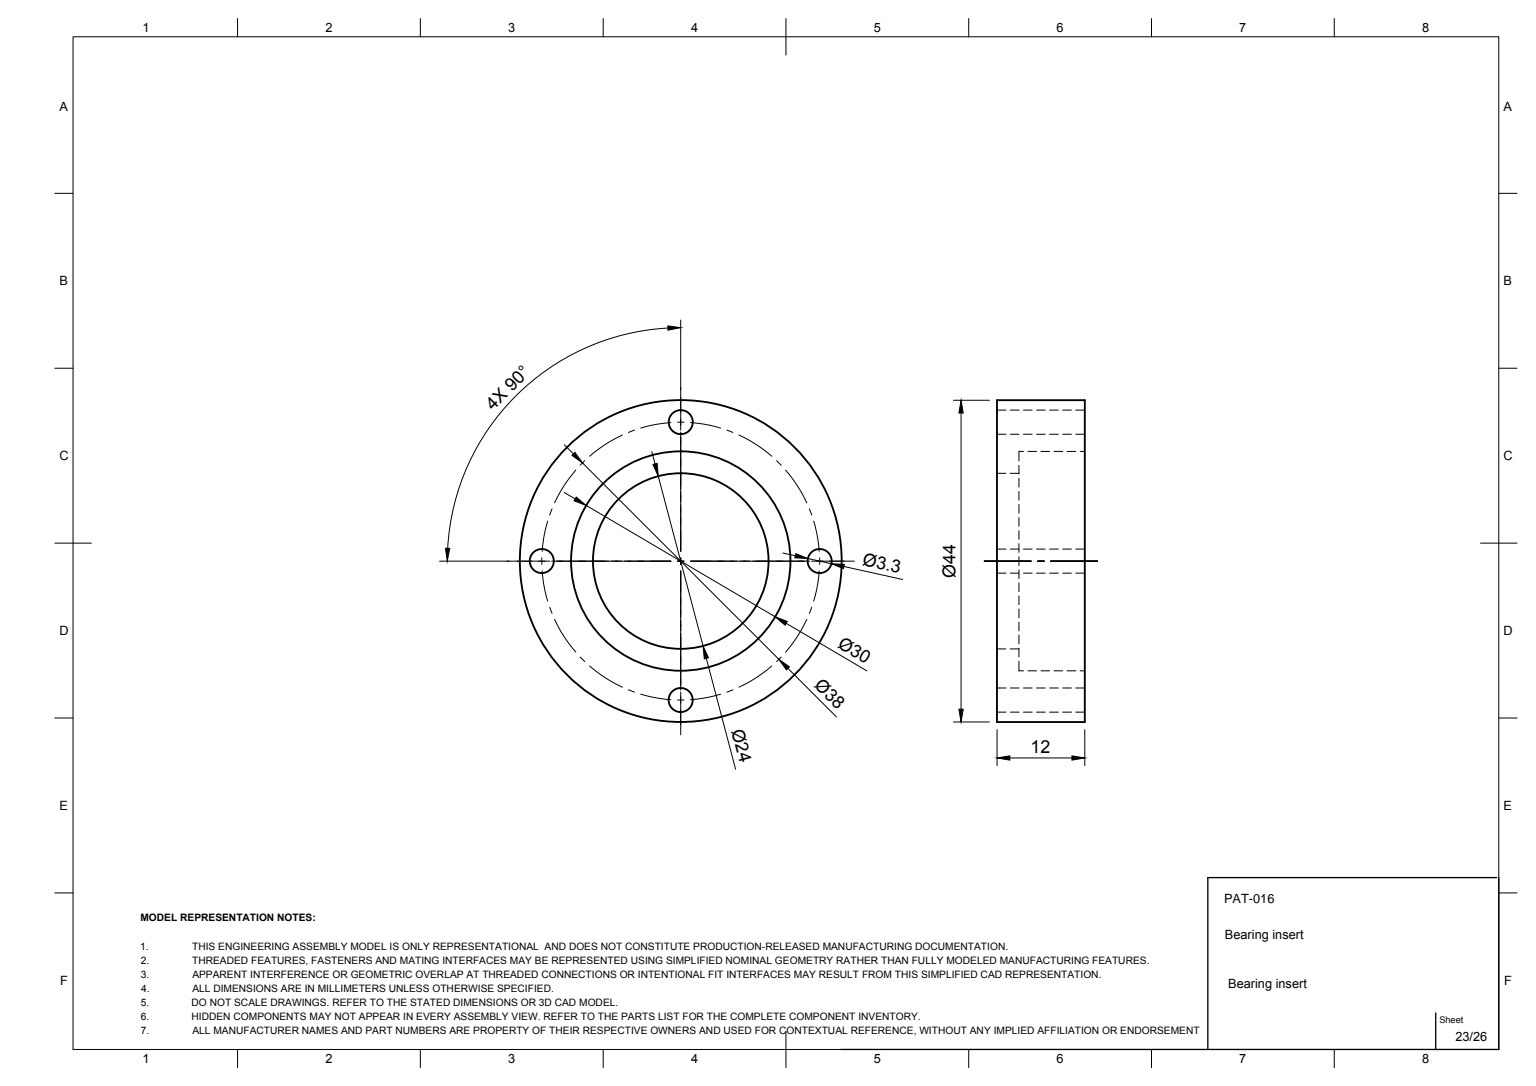
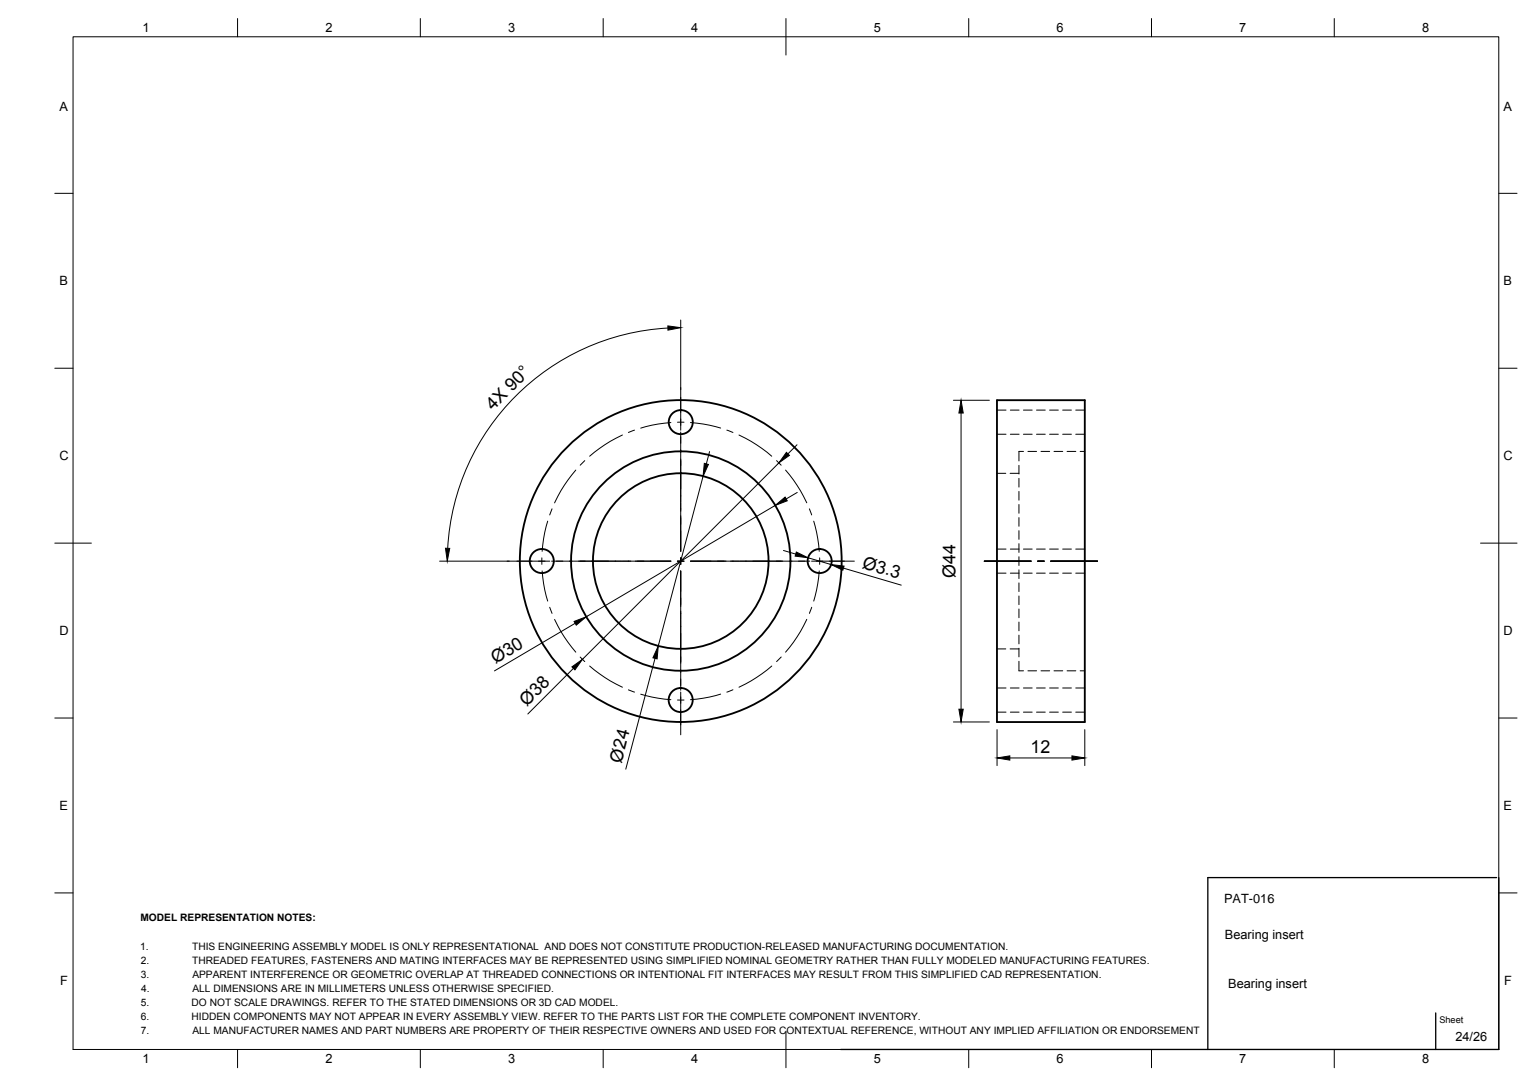
ISO-10303-21;
HEADER;
/* Generated by software containing ST-Developer
 * from STEP Tools, Inc. (www.steptools.com) 
 */

FILE_DESCRIPTION(
/* description */ ('Bracket-mounted idler roller'),
/* implementation_level */ '2;1');

FILE_NAME(
/* name */ 'Bearing insert.step',
/* time_stamp */ '2026-10-28T03:26:42-07:00',
/* author */ (''),
/* organization */ (''),
/* preprocessor_version */ 'ST-DEVELOPER v20.2',
/* originating_system */ 'Autodesk Translation Framework v15.17.0.0',
/* authorisation */ '');

FILE_SCHEMA (('AUTOMOTIVE_DESIGN { 1 0 10303 214 3 1 1 }'));
ENDSEC;

DATA;
#10=MECHANICAL_DESIGN_GEOMETRIC_PRESENTATION_REPRESENTATION('',(#304),#6241);
#254=SHAPE_REPRESENTATION_RELATIONSHIP('SRR','None',#6360,#275);
#275=ADVANCED_BREP_SHAPE_REPRESENTATION('',(#332),#6236);
#304=STYLED_ITEM('',(#6538),#332);
#332=MANIFOLD_SOLID_BREP('Body1',#3207);
#382=FACE_BOUND('',#901,.T.);
#383=FACE_BOUND('',#905,.T.);
#384=FACE_BOUND('',#906,.T.);
#385=FACE_BOUND('',#907,.T.);
#386=FACE_BOUND('',#908,.T.);
#387=FACE_BOUND('',#909,.T.);
#388=FACE_BOUND('',#911,.T.);
#389=FACE_BOUND('',#912,.T.);
#390=FACE_BOUND('',#913,.T.);
#391=FACE_BOUND('',#914,.T.);
#392=FACE_BOUND('',#915,.T.);
#495=PLANE('',#3757);
#496=PLANE('',#3764);
#497=PLANE('',#3765);
#658=FACE_OUTER_BOUND('',#895,.T.);
#659=FACE_OUTER_BOUND('',#896,.T.);
#660=FACE_OUTER_BOUND('',#897,.T.);
#661=FACE_OUTER_BOUND('',#898,.T.);
#662=FACE_OUTER_BOUND('',#899,.T.);
#663=FACE_OUTER_BOUND('',#900,.T.);
#664=FACE_OUTER_BOUND('',#902,.T.);
#665=FACE_OUTER_BOUND('',#903,.T.);
#666=FACE_OUTER_BOUND('',#904,.T.);
#667=FACE_OUTER_BOUND('',#910,.T.);
#895=EDGE_LOOP('',(#2732,#2733,#2734,#2735));
#896=EDGE_LOOP('',(#2736,#2737,#2738,#2739));
#897=EDGE_LOOP('',(#2740,#2741,#2742,#2743));
#898=EDGE_LOOP('',(#2744,#2745,#2746,#2747));
#899=EDGE_LOOP('',(#2748,#2749,#2750,#2751));
#900=EDGE_LOOP('',(#2752));
#901=EDGE_LOOP('',(#2753));
#902=EDGE_LOOP('',(#2754,#2755,#2756,#2757));
#903=EDGE_LOOP('',(#2758,#2759,#2760,#2761));
#904=EDGE_LOOP('',(#2762));
#905=EDGE_LOOP('',(#2763));
#906=EDGE_LOOP('',(#2764));
#907=EDGE_LOOP('',(#2765));
#908=EDGE_LOOP('',(#2766));
#909=EDGE_LOOP('',(#2767));
#910=EDGE_LOOP('',(#2768));
#911=EDGE_LOOP('',(#2769));
#912=EDGE_LOOP('',(#2770));
#913=EDGE_LOOP('',(#2771));
#914=EDGE_LOOP('',(#2772));
#915=EDGE_LOOP('',(#2773));
#1115=LINE('',#5940,#1297);
#1116=LINE('',#5946,#1298);
#1117=LINE('',#5952,#1299);
#1118=LINE('',#5958,#1300);
#1119=LINE('',#5964,#1301);
#1120=LINE('',#5971,#1302);
#1121=LINE('',#5977,#1303);
#1297=VECTOR('',#4620,0.165);
#1298=VECTOR('',#4627,0.165);
#1299=VECTOR('',#4634,0.165);
#1300=VECTOR('',#4641,0.165);
#1301=VECTOR('',#4648,1.2);
#1302=VECTOR('',#4657,1.5);
#1303=VECTOR('',#4664,2.2);
#1472=CIRCLE('',#3743,0.165);
#1473=CIRCLE('',#3744,0.165);
#1474=CIRCLE('',#3746,0.165);
#1475=CIRCLE('',#3747,0.165);
#1476=CIRCLE('',#3749,0.165);
#1477=CIRCLE('',#3750,0.165);
#1478=CIRCLE('',#3752,0.165);
#1479=CIRCLE('',#3753,0.165);
#1480=CIRCLE('',#3755,1.2);
#1481=CIRCLE('',#3756,1.2);
#1482=CIRCLE('',#3758,1.5);
#1483=CIRCLE('',#3760,1.5);
#1484=CIRCLE('',#3762,2.2);
#1485=CIRCLE('',#3763,2.2);
#1721=VERTEX_POINT('',#5937);
#1722=VERTEX_POINT('',#5939);
#1723=VERTEX_POINT('',#5943);
#1724=VERTEX_POINT('',#5945);
#1725=VERTEX_POINT('',#5949);
#1726=VERTEX_POINT('',#5951);
#1727=VERTEX_POINT('',#5955);
#1728=VERTEX_POINT('',#5957);
#1729=VERTEX_POINT('',#5961);
#1730=VERTEX_POINT('',#5963);
#1731=VERTEX_POINT('',#5967);
#1732=VERTEX_POINT('',#5970);
#1733=VERTEX_POINT('',#5974);
#1734=VERTEX_POINT('',#5976);
#2068=EDGE_CURVE('',#1721,#1721,#1472,.T.);
#2069=EDGE_CURVE('',#1721,#1722,#1115,.T.);
#2070=EDGE_CURVE('',#1722,#1722,#1473,.T.);
#2071=EDGE_CURVE('',#1723,#1723,#1474,.T.);
#2072=EDGE_CURVE('',#1723,#1724,#1116,.T.);
#2073=EDGE_CURVE('',#1724,#1724,#1475,.T.);
#2074=EDGE_CURVE('',#1725,#1725,#1476,.T.);
#2075=EDGE_CURVE('',#1725,#1726,#1117,.T.);
#2076=EDGE_CURVE('',#1726,#1726,#1477,.T.);
#2077=EDGE_CURVE('',#1727,#1727,#1478,.T.);
#2078=EDGE_CURVE('',#1727,#1728,#1118,.T.);
#2079=EDGE_CURVE('',#1728,#1728,#1479,.T.);
#2080=EDGE_CURVE('',#1729,#1729,#1480,.T.);
#2081=EDGE_CURVE('',#1729,#1730,#1119,.T.);
#2082=EDGE_CURVE('',#1730,#1730,#1481,.T.);
#2083=EDGE_CURVE('',#1731,#1731,#1482,.T.);
#2084=EDGE_CURVE('',#1731,#1732,#1120,.T.);
#2085=EDGE_CURVE('',#1732,#1732,#1483,.T.);
#2086=EDGE_CURVE('',#1733,#1733,#1484,.T.);
#2087=EDGE_CURVE('',#1733,#1734,#1121,.T.);
#2088=EDGE_CURVE('',#1734,#1734,#1485,.T.);
#2732=ORIENTED_EDGE('',*,*,#2068,.F.);
#2733=ORIENTED_EDGE('',*,*,#2069,.T.);
#2734=ORIENTED_EDGE('',*,*,#2070,.F.);
#2735=ORIENTED_EDGE('',*,*,#2069,.F.);
#2736=ORIENTED_EDGE('',*,*,#2071,.F.);
#2737=ORIENTED_EDGE('',*,*,#2072,.T.);
#2738=ORIENTED_EDGE('',*,*,#2073,.F.);
#2739=ORIENTED_EDGE('',*,*,#2072,.F.);
#2740=ORIENTED_EDGE('',*,*,#2074,.F.);
#2741=ORIENTED_EDGE('',*,*,#2075,.T.);
#2742=ORIENTED_EDGE('',*,*,#2076,.F.);
#2743=ORIENTED_EDGE('',*,*,#2075,.F.);
#2744=ORIENTED_EDGE('',*,*,#2077,.F.);
#2745=ORIENTED_EDGE('',*,*,#2078,.T.);
#2746=ORIENTED_EDGE('',*,*,#2079,.F.);
#2747=ORIENTED_EDGE('',*,*,#2078,.F.);
#2748=ORIENTED_EDGE('',*,*,#2080,.F.);
#2749=ORIENTED_EDGE('',*,*,#2081,.T.);
#2750=ORIENTED_EDGE('',*,*,#2082,.T.);
#2751=ORIENTED_EDGE('',*,*,#2081,.F.);
#2752=ORIENTED_EDGE('',*,*,#2083,.F.);
#2753=ORIENTED_EDGE('',*,*,#2082,.F.);
#2754=ORIENTED_EDGE('',*,*,#2083,.T.);
#2755=ORIENTED_EDGE('',*,*,#2084,.T.);
#2756=ORIENTED_EDGE('',*,*,#2085,.T.);
#2757=ORIENTED_EDGE('',*,*,#2084,.F.);
#2758=ORIENTED_EDGE('',*,*,#2086,.F.);
#2759=ORIENTED_EDGE('',*,*,#2087,.T.);
#2760=ORIENTED_EDGE('',*,*,#2088,.T.);
#2761=ORIENTED_EDGE('',*,*,#2087,.F.);
#2762=ORIENTED_EDGE('',*,*,#2086,.T.);
#2763=ORIENTED_EDGE('',*,*,#2080,.T.);
#2764=ORIENTED_EDGE('',*,*,#2079,.T.);
#2765=ORIENTED_EDGE('',*,*,#2076,.T.);
#2766=ORIENTED_EDGE('',*,*,#2073,.T.);
#2767=ORIENTED_EDGE('',*,*,#2070,.T.);
#2768=ORIENTED_EDGE('',*,*,#2088,.F.);
#2769=ORIENTED_EDGE('',*,*,#2085,.F.);
#2770=ORIENTED_EDGE('',*,*,#2077,.T.);
#2771=ORIENTED_EDGE('',*,*,#2074,.T.);
#2772=ORIENTED_EDGE('',*,*,#2071,.T.);
#2773=ORIENTED_EDGE('',*,*,#2068,.T.);
#2967=CYLINDRICAL_SURFACE('',#3742,0.165);
#2968=CYLINDRICAL_SURFACE('',#3745,0.165);
#2969=CYLINDRICAL_SURFACE('',#3748,0.165);
#2970=CYLINDRICAL_SURFACE('',#3751,0.165);
#2971=CYLINDRICAL_SURFACE('',#3754,1.2);
#2972=CYLINDRICAL_SURFACE('',#3759,1.5);
#2973=CYLINDRICAL_SURFACE('',#3761,2.2);
#3133=ADVANCED_FACE('',(#658),#2967,.F.);
#3134=ADVANCED_FACE('',(#659),#2968,.F.);
#3135=ADVANCED_FACE('',(#660),#2969,.F.);
#3136=ADVANCED_FACE('',(#661),#2970,.F.);
#3137=ADVANCED_FACE('',(#662),#2971,.F.);
#3138=ADVANCED_FACE('',(#663,#382),#495,.F.);
#3139=ADVANCED_FACE('',(#664),#2972,.F.);
#3140=ADVANCED_FACE('',(#665),#2973,.T.);
#3141=ADVANCED_FACE('',(#666,#383,#384,#385,#386,#387),#496,.T.);
#3142=ADVANCED_FACE('',(#667,#388,#389,#390,#391,#392),#497,.F.);
#3207=CLOSED_SHELL('',(#3133,#3134,#3135,#3136,#3137,#3138,#3139,#3140,
#3141,#3142));
#3741=AXIS2_PLACEMENT_3D('',#5935,#4614,#4615);
#3742=AXIS2_PLACEMENT_3D('',#5936,#4616,#4617);
#3743=AXIS2_PLACEMENT_3D('',#5938,#4618,#4619);
#3744=AXIS2_PLACEMENT_3D('',#5941,#4621,#4622);
#3745=AXIS2_PLACEMENT_3D('',#5942,#4623,#4624);
#3746=AXIS2_PLACEMENT_3D('',#5944,#4625,#4626);
#3747=AXIS2_PLACEMENT_3D('',#5947,#4628,#4629);
#3748=AXIS2_PLACEMENT_3D('',#5948,#4630,#4631);
#3749=AXIS2_PLACEMENT_3D('',#5950,#4632,#4633);
#3750=AXIS2_PLACEMENT_3D('',#5953,#4635,#4636);
#3751=AXIS2_PLACEMENT_3D('',#5954,#4637,#4638);
#3752=AXIS2_PLACEMENT_3D('',#5956,#4639,#4640);
#3753=AXIS2_PLACEMENT_3D('',#5959,#4642,#4643);
#3754=AXIS2_PLACEMENT_3D('',#5960,#4644,#4645);
#3755=AXIS2_PLACEMENT_3D('',#5962,#4646,#4647);
#3756=AXIS2_PLACEMENT_3D('',#5965,#4649,#4650);
#3757=AXIS2_PLACEMENT_3D('',#5966,#4651,#4652);
#3758=AXIS2_PLACEMENT_3D('',#5968,#4653,#4654);
#3759=AXIS2_PLACEMENT_3D('',#5969,#4655,#4656);
#3760=AXIS2_PLACEMENT_3D('',#5972,#4658,#4659);
#3761=AXIS2_PLACEMENT_3D('',#5973,#4660,#4661);
#3762=AXIS2_PLACEMENT_3D('',#5975,#4662,#4663);
#3763=AXIS2_PLACEMENT_3D('',#5978,#4665,#4666);
#3764=AXIS2_PLACEMENT_3D('',#5979,#4667,#4668);
#3765=AXIS2_PLACEMENT_3D('',#5980,#4669,#4670);
#4614=DIRECTION('axis',(0.,0.,1.));
#4615=DIRECTION('refdir',(1.,0.,0.));
#4616=DIRECTION('center_axis',(0.,1.,0.));
#4617=DIRECTION('ref_axis',(1.,0.,0.));
#4618=DIRECTION('center_axis',(0.,1.,0.));
#4619=DIRECTION('ref_axis',(1.,0.,0.));
#4620=DIRECTION('',(0.,1.,0.));
#4621=DIRECTION('center_axis',(0.,-1.,0.));
#4622=DIRECTION('ref_axis',(1.,0.,0.));
#4623=DIRECTION('center_axis',(0.,1.,0.));
#4624=DIRECTION('ref_axis',(1.,0.,0.));
#4625=DIRECTION('center_axis',(0.,1.,0.));
#4626=DIRECTION('ref_axis',(1.,0.,0.));
#4627=DIRECTION('',(0.,1.,0.));
#4628=DIRECTION('center_axis',(0.,-1.,0.));
#4629=DIRECTION('ref_axis',(1.,0.,0.));
#4630=DIRECTION('center_axis',(0.,1.,0.));
#4631=DIRECTION('ref_axis',(1.,0.,0.));
#4632=DIRECTION('center_axis',(0.,1.,0.));
#4633=DIRECTION('ref_axis',(1.,0.,0.));
#4634=DIRECTION('',(0.,1.,0.));
#4635=DIRECTION('center_axis',(0.,-1.,0.));
#4636=DIRECTION('ref_axis',(1.,0.,0.));
#4637=DIRECTION('center_axis',(0.,1.,0.));
#4638=DIRECTION('ref_axis',(1.,0.,0.));
#4639=DIRECTION('center_axis',(0.,1.,0.));
#4640=DIRECTION('ref_axis',(1.,0.,0.));
#4641=DIRECTION('',(0.,1.,0.));
#4642=DIRECTION('center_axis',(0.,-1.,0.));
#4643=DIRECTION('ref_axis',(1.,0.,0.));
#4644=DIRECTION('center_axis',(0.,1.,0.));
#4645=DIRECTION('ref_axis',(1.,0.,0.));
#4646=DIRECTION('center_axis',(0.,-1.,0.));
#4647=DIRECTION('ref_axis',(1.,0.,0.));
#4648=DIRECTION('',(0.,-1.,0.));
#4649=DIRECTION('center_axis',(0.,-1.,0.));
#4650=DIRECTION('ref_axis',(1.,0.,0.));
#4651=DIRECTION('center_axis',(0.,1.,0.));
#4652=DIRECTION('ref_axis',(1.,0.,0.));
#4653=DIRECTION('center_axis',(0.,1.,0.));
#4654=DIRECTION('ref_axis',(1.,0.,0.));
#4655=DIRECTION('center_axis',(0.,1.,0.));
#4656=DIRECTION('ref_axis',(1.,0.,0.));
#4657=DIRECTION('',(0.,-1.,0.));
#4658=DIRECTION('center_axis',(0.,-1.,0.));
#4659=DIRECTION('ref_axis',(1.,0.,0.));
#4660=DIRECTION('center_axis',(0.,1.,0.));
#4661=DIRECTION('ref_axis',(1.,0.,0.));
#4662=DIRECTION('center_axis',(0.,1.,0.));
#4663=DIRECTION('ref_axis',(1.,0.,0.));
#4664=DIRECTION('',(0.,-1.,0.));
#4665=DIRECTION('center_axis',(0.,1.,0.));
#4666=DIRECTION('ref_axis',(1.,0.,0.));
#4667=DIRECTION('center_axis',(0.,1.,0.));
#4668=DIRECTION('ref_axis',(1.,0.,0.));
#4669=DIRECTION('center_axis',(0.,1.,0.));
#4670=DIRECTION('ref_axis',(1.,0.,0.));
#5935=CARTESIAN_POINT('',(0.,0.,0.));
#5936=CARTESIAN_POINT('Origin',(-1.9,-0.1,4.5));
#5937=CARTESIAN_POINT('',(-2.065,0.,4.5));
#5938=CARTESIAN_POINT('Origin',(-1.9,0.,4.5));
#5939=CARTESIAN_POINT('',(-2.065,1.2,4.5));
#5940=CARTESIAN_POINT('',(-2.065,-0.1,4.5));
#5941=CARTESIAN_POINT('Origin',(-1.9,1.2,4.5));
#5942=CARTESIAN_POINT('Origin',(1.16341445918999E-16,-0.1,6.4));
#5943=CARTESIAN_POINT('',(-0.165,0.,6.4));
#5944=CARTESIAN_POINT('Origin',(1.16341445918999E-16,0.,6.4));
#5945=CARTESIAN_POINT('',(-0.165,1.2,6.4));
#5946=CARTESIAN_POINT('',(-0.165,-0.1,6.4));
#5947=CARTESIAN_POINT('Origin',(1.16341445918999E-16,1.2,6.4));
#5948=CARTESIAN_POINT('Origin',(1.9,-0.1,4.5));
#5949=CARTESIAN_POINT('',(1.735,0.,4.5));
#5950=CARTESIAN_POINT('Origin',(1.9,0.,4.5));
#5951=CARTESIAN_POINT('',(1.735,1.2,4.5));
#5952=CARTESIAN_POINT('',(1.735,-0.1,4.5));
#5953=CARTESIAN_POINT('Origin',(1.9,1.2,4.5));
#5954=CARTESIAN_POINT('Origin',(-3.49024337756996E-16,-0.1,2.6));
#5955=CARTESIAN_POINT('',(-0.165,0.,2.6));
#5956=CARTESIAN_POINT('Origin',(-3.49024337756996E-16,0.,2.6));
#5957=CARTESIAN_POINT('',(-0.165,1.2,2.6));
#5958=CARTESIAN_POINT('',(-0.165,-0.1,2.6));
#5959=CARTESIAN_POINT('Origin',(-3.49024337756996E-16,1.2,2.6));
#5960=CARTESIAN_POINT('Origin',(0.,0.9,4.5));
#5961=CARTESIAN_POINT('',(-1.2,1.2,4.5));
#5962=CARTESIAN_POINT('Origin',(0.,1.2,4.5));
#5963=CARTESIAN_POINT('',(-1.2,0.9,4.5));
#5964=CARTESIAN_POINT('',(-1.2,0.9,4.5));
#5965=CARTESIAN_POINT('Origin',(0.,0.9,4.5));
#5966=CARTESIAN_POINT('Origin',(0.,0.9,4.5));
#5967=CARTESIAN_POINT('',(-1.5,0.9,4.5));
#5968=CARTESIAN_POINT('Origin',(0.,0.9,4.5));
#5969=CARTESIAN_POINT('Origin',(0.,0.,4.5));
#5970=CARTESIAN_POINT('',(-1.5,0.,4.5));
#5971=CARTESIAN_POINT('',(-1.5,0.,4.5));
#5972=CARTESIAN_POINT('Origin',(0.,0.,4.5));
#5973=CARTESIAN_POINT('Origin',(0.,0.,4.5));
#5974=CARTESIAN_POINT('',(-2.2,1.2,4.5));
#5975=CARTESIAN_POINT('Origin',(0.,1.2,4.5));
#5976=CARTESIAN_POINT('',(-2.2,0.,4.5));
#5977=CARTESIAN_POINT('',(-2.2,0.,4.5));
#5978=CARTESIAN_POINT('Origin',(0.,0.,4.5));
#5979=CARTESIAN_POINT('Origin',(0.,1.2,4.5));
#5980=CARTESIAN_POINT('Origin',(0.,0.,4.5));
#6210=UNCERTAINTY_MEASURE_WITH_UNIT(LENGTH_MEASURE(0.001),#6242,
'DISTANCE_ACCURACY_VALUE',
'Maximum model space distance between geometric entities at asserted c
onnectivities');
#6215=UNCERTAINTY_MEASURE_WITH_UNIT(LENGTH_MEASURE(0.001),#6242,
'DISTANCE_ACCURACY_VALUE',
'Maximum model space distance between geometric entities at asserted c
onnectivities');
#6236=(
GEOMETRIC_REPRESENTATION_CONTEXT(3)
GLOBAL_UNCERTAINTY_ASSIGNED_CONTEXT((#6210))
GLOBAL_UNIT_ASSIGNED_CONTEXT((#6242,#6244,#6245))
REPRESENTATION_CONTEXT('','3D')
);
#6241=(
GEOMETRIC_REPRESENTATION_CONTEXT(3)
GLOBAL_UNCERTAINTY_ASSIGNED_CONTEXT((#6215))
GLOBAL_UNIT_ASSIGNED_CONTEXT((#6242,#6244,#6245))
REPRESENTATION_CONTEXT('','3D')
);
#6242=(
LENGTH_UNIT()
NAMED_UNIT(*)
SI_UNIT(.CENTI.,.METRE.)
);
#6244=(
NAMED_UNIT(*)
PLANE_ANGLE_UNIT()
SI_UNIT($,.RADIAN.)
);
#6245=(
NAMED_UNIT(*)
SI_UNIT($,.STERADIAN.)
SOLID_ANGLE_UNIT()
);
#6266=SHAPE_DEFINITION_REPRESENTATION(#6296,#6360);
#6296=PRODUCT_DEFINITION_SHAPE('',$,#6386);
#6360=SHAPE_REPRESENTATION('',(#3741),#6236);
#6365=PRODUCT_DEFINITION_CONTEXT('part definition',#6442,'design');
#6386=PRODUCT_DEFINITION('Bearing insert','Bearing insert',#6411,#6365);
#6411=PRODUCT_DEFINITION_FORMATION('',$,#6464);
#6442=APPLICATION_CONTEXT(
'Core Data for Automotive Mechanical Design Process');
#6443=PRODUCT_CONTEXT('part definition',#6442,'mechanical');
#6464=PRODUCT('Bearing insert','Bearing insert','Bearing insert',(#6443));
#6532=COLOUR_RGB('Grey',0.48,0.52,0.57);
#6533=FILL_AREA_STYLE_COLOUR('',#6532);
#6534=FILL_AREA_STYLE('',(#6533));
#6535=SURFACE_STYLE_FILL_AREA(#6534);
#6536=SURFACE_SIDE_STYLE('',(#6535));
#6537=SURFACE_STYLE_USAGE(.BOTH.,#6536);
#6538=PRESENTATION_STYLE_ASSIGNMENT((#6537));
ENDSEC;
END-ISO-10303-21;
